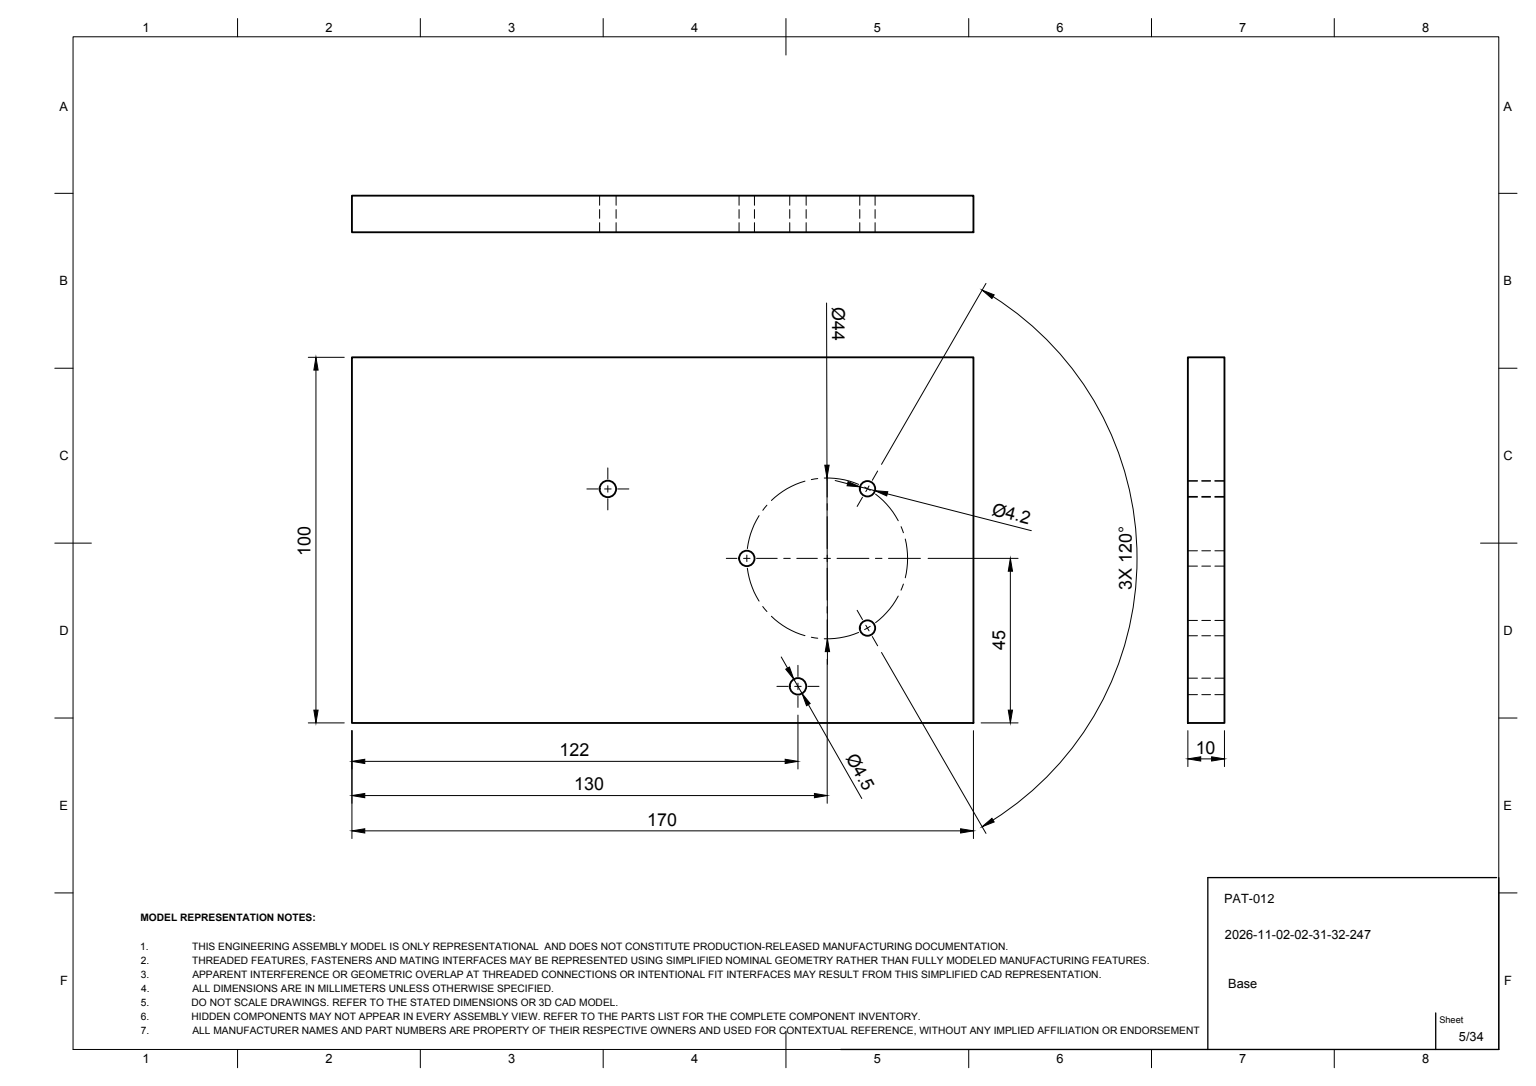
ISO-10303-21;
HEADER;
/* Generated by software containing ST-Developer
 * from STEP Tools, Inc. (www.steptools.com) 
 */

FILE_DESCRIPTION(
/* description */ ('Belt tensioner idler arm'),
/* implementation_level */ '2;1');

FILE_NAME(
/* name */ 'Base.step',
/* time_stamp */ '2026-10-28T03:22:15-07:00',
/* author */ (''),
/* organization */ (''),
/* preprocessor_version */ 'ST-DEVELOPER v20.2',
/* originating_system */ 'Autodesk Translation Framework v15.17.0.0',
/* authorisation */ '');

FILE_SCHEMA (('AUTOMOTIVE_DESIGN { 1 0 10303 214 3 1 1 }'));
ENDSEC;

DATA;
#10=MECHANICAL_DESIGN_GEOMETRIC_PRESENTATION_REPRESENTATION('',(#447),#12779);
#379=SHAPE_REPRESENTATION_RELATIONSHIP('SRR','None',#12925,#413);
#413=ADVANCED_BREP_SHAPE_REPRESENTATION('',(#489),#12742);
#447=STYLED_ITEM('',(#13163),#489);
#489=MANIFOLD_SOLID_BREP('Body1',#6181);
#527=FACE_BOUND('',#1214,.T.);
#528=FACE_BOUND('',#1215,.T.);
#529=FACE_BOUND('',#1216,.T.);
#530=FACE_BOUND('',#1217,.T.);
#531=FACE_BOUND('',#1218,.T.);
#532=FACE_BOUND('',#1220,.T.);
#533=FACE_BOUND('',#1221,.T.);
#534=FACE_BOUND('',#1222,.T.);
#535=FACE_BOUND('',#1223,.T.);
#536=FACE_BOUND('',#1224,.T.);
#663=PLANE('',#6620);
#664=PLANE('',#6621);
#665=PLANE('',#6622);
#666=PLANE('',#6623);
#667=PLANE('',#6624);
#668=PLANE('',#6625);
#837=FACE_OUTER_BOUND('',#1204,.T.);
#838=FACE_OUTER_BOUND('',#1205,.T.);
#839=FACE_OUTER_BOUND('',#1206,.T.);
#840=FACE_OUTER_BOUND('',#1207,.T.);
#841=FACE_OUTER_BOUND('',#1208,.T.);
#842=FACE_OUTER_BOUND('',#1209,.T.);
#843=FACE_OUTER_BOUND('',#1210,.T.);
#844=FACE_OUTER_BOUND('',#1211,.T.);
#845=FACE_OUTER_BOUND('',#1212,.T.);
#846=FACE_OUTER_BOUND('',#1213,.T.);
#847=FACE_OUTER_BOUND('',#1219,.T.);
#1204=EDGE_LOOP('',(#4086,#4087,#4088,#4089));
#1205=EDGE_LOOP('',(#4090,#4091,#4092,#4093));
#1206=EDGE_LOOP('',(#4094,#4095,#4096,#4097));
#1207=EDGE_LOOP('',(#4098,#4099,#4100,#4101));
#1208=EDGE_LOOP('',(#4102,#4103,#4104,#4105));
#1209=EDGE_LOOP('',(#4106,#4107,#4108,#4109));
#1210=EDGE_LOOP('',(#4110,#4111,#4112,#4113));
#1211=EDGE_LOOP('',(#4114,#4115,#4116,#4117));
#1212=EDGE_LOOP('',(#4118,#4119,#4120,#4121));
#1213=EDGE_LOOP('',(#4122,#4123,#4124,#4125));
#1214=EDGE_LOOP('',(#4126));
#1215=EDGE_LOOP('',(#4127));
#1216=EDGE_LOOP('',(#4128));
#1217=EDGE_LOOP('',(#4129));
#1218=EDGE_LOOP('',(#4130));
#1219=EDGE_LOOP('',(#4131,#4132,#4133,#4134));
#1220=EDGE_LOOP('',(#4135));
#1221=EDGE_LOOP('',(#4136));
#1222=EDGE_LOOP('',(#4137));
#1223=EDGE_LOOP('',(#4138));
#1224=EDGE_LOOP('',(#4139));
#1707=LINE('',#9451,#2056);
#1708=LINE('',#9457,#2057);
#1709=LINE('',#9463,#2058);
#1710=LINE('',#9469,#2059);
#1711=LINE('',#9475,#2060);
#1712=LINE('',#9480,#2061);
#1713=LINE('',#9482,#2062);
#1714=LINE('',#9484,#2063);
#1715=LINE('',#9485,#2064);
#1716=LINE('',#9488,#2065);
#1717=LINE('',#9490,#2066);
#1718=LINE('',#9491,#2067);
#1719=LINE('',#9494,#2068);
#1720=LINE('',#9496,#2069);
#1721=LINE('',#9497,#2070);
#1722=LINE('',#9499,#2071);
#1723=LINE('',#9500,#2072);
#2056=VECTOR('',#7443,0.225);
#2057=VECTOR('',#7450,0.225);
#2058=VECTOR('',#7457,0.21);
#2059=VECTOR('',#7464,0.21);
#2060=VECTOR('',#7471,0.21);
#2061=VECTOR('',#7476,1.);
#2062=VECTOR('',#7477,1.);
#2063=VECTOR('',#7478,1.);
#2064=VECTOR('',#7479,1.);
#2065=VECTOR('',#7482,1.);
#2066=VECTOR('',#7483,1.);
#2067=VECTOR('',#7484,1.);
#2068=VECTOR('',#7487,1.);
#2069=VECTOR('',#7488,1.);
#2070=VECTOR('',#7489,1.);
#2071=VECTOR('',#7492,1.);
#2072=VECTOR('',#7493,1.);
#2405=CIRCLE('',#6606,0.225);
#2406=CIRCLE('',#6607,0.225);
#2407=CIRCLE('',#6609,0.225);
#2408=CIRCLE('',#6610,0.225);
#2409=CIRCLE('',#6612,0.21);
#2410=CIRCLE('',#6613,0.21);
#2411=CIRCLE('',#6615,0.21);
#2412=CIRCLE('',#6616,0.21);
#2413=CIRCLE('',#6618,0.21);
#2414=CIRCLE('',#6619,0.21);
#2769=VERTEX_POINT('',#9448);
#2770=VERTEX_POINT('',#9450);
#2771=VERTEX_POINT('',#9454);
#2772=VERTEX_POINT('',#9456);
#2773=VERTEX_POINT('',#9460);
#2774=VERTEX_POINT('',#9462);
#2775=VERTEX_POINT('',#9466);
#2776=VERTEX_POINT('',#9468);
#2777=VERTEX_POINT('',#9472);
#2778=VERTEX_POINT('',#9474);
#2779=VERTEX_POINT('',#9478);
#2780=VERTEX_POINT('',#9479);
#2781=VERTEX_POINT('',#9481);
#2782=VERTEX_POINT('',#9483);
#2783=VERTEX_POINT('',#9487);
#2784=VERTEX_POINT('',#9489);
#2785=VERTEX_POINT('',#9493);
#2786=VERTEX_POINT('',#9495);
#3298=EDGE_CURVE('',#2769,#2769,#2405,.T.);
#3299=EDGE_CURVE('',#2769,#2770,#1707,.T.);
#3300=EDGE_CURVE('',#2770,#2770,#2406,.T.);
#3301=EDGE_CURVE('',#2771,#2771,#2407,.T.);
#3302=EDGE_CURVE('',#2771,#2772,#1708,.T.);
#3303=EDGE_CURVE('',#2772,#2772,#2408,.T.);
#3304=EDGE_CURVE('',#2773,#2773,#2409,.T.);
#3305=EDGE_CURVE('',#2773,#2774,#1709,.T.);
#3306=EDGE_CURVE('',#2774,#2774,#2410,.T.);
#3307=EDGE_CURVE('',#2775,#2775,#2411,.T.);
#3308=EDGE_CURVE('',#2775,#2776,#1710,.T.);
#3309=EDGE_CURVE('',#2776,#2776,#2412,.T.);
#3310=EDGE_CURVE('',#2777,#2777,#2413,.T.);
#3311=EDGE_CURVE('',#2777,#2778,#1711,.T.);
#3312=EDGE_CURVE('',#2778,#2778,#2414,.T.);
#3313=EDGE_CURVE('',#2779,#2780,#1712,.T.);
#3314=EDGE_CURVE('',#2780,#2781,#1713,.T.);
#3315=EDGE_CURVE('',#2782,#2781,#1714,.T.);
#3316=EDGE_CURVE('',#2779,#2782,#1715,.T.);
#3317=EDGE_CURVE('',#2783,#2779,#1716,.T.);
#3318=EDGE_CURVE('',#2784,#2782,#1717,.T.);
#3319=EDGE_CURVE('',#2783,#2784,#1718,.T.);
#3320=EDGE_CURVE('',#2785,#2783,#1719,.T.);
#3321=EDGE_CURVE('',#2786,#2784,#1720,.T.);
#3322=EDGE_CURVE('',#2785,#2786,#1721,.T.);
#3323=EDGE_CURVE('',#2780,#2785,#1722,.T.);
#3324=EDGE_CURVE('',#2781,#2786,#1723,.T.);
#4086=ORIENTED_EDGE('',*,*,#3298,.F.);
#4087=ORIENTED_EDGE('',*,*,#3299,.T.);
#4088=ORIENTED_EDGE('',*,*,#3300,.F.);
#4089=ORIENTED_EDGE('',*,*,#3299,.F.);
#4090=ORIENTED_EDGE('',*,*,#3301,.F.);
#4091=ORIENTED_EDGE('',*,*,#3302,.T.);
#4092=ORIENTED_EDGE('',*,*,#3303,.F.);
#4093=ORIENTED_EDGE('',*,*,#3302,.F.);
#4094=ORIENTED_EDGE('',*,*,#3304,.F.);
#4095=ORIENTED_EDGE('',*,*,#3305,.T.);
#4096=ORIENTED_EDGE('',*,*,#3306,.F.);
#4097=ORIENTED_EDGE('',*,*,#3305,.F.);
#4098=ORIENTED_EDGE('',*,*,#3307,.F.);
#4099=ORIENTED_EDGE('',*,*,#3308,.T.);
#4100=ORIENTED_EDGE('',*,*,#3309,.F.);
#4101=ORIENTED_EDGE('',*,*,#3308,.F.);
#4102=ORIENTED_EDGE('',*,*,#3310,.F.);
#4103=ORIENTED_EDGE('',*,*,#3311,.T.);
#4104=ORIENTED_EDGE('',*,*,#3312,.F.);
#4105=ORIENTED_EDGE('',*,*,#3311,.F.);
#4106=ORIENTED_EDGE('',*,*,#3313,.T.);
#4107=ORIENTED_EDGE('',*,*,#3314,.T.);
#4108=ORIENTED_EDGE('',*,*,#3315,.F.);
#4109=ORIENTED_EDGE('',*,*,#3316,.F.);
#4110=ORIENTED_EDGE('',*,*,#3317,.T.);
#4111=ORIENTED_EDGE('',*,*,#3316,.T.);
#4112=ORIENTED_EDGE('',*,*,#3318,.F.);
#4113=ORIENTED_EDGE('',*,*,#3319,.F.);
#4114=ORIENTED_EDGE('',*,*,#3320,.T.);
#4115=ORIENTED_EDGE('',*,*,#3319,.T.);
#4116=ORIENTED_EDGE('',*,*,#3321,.F.);
#4117=ORIENTED_EDGE('',*,*,#3322,.F.);
#4118=ORIENTED_EDGE('',*,*,#3323,.T.);
#4119=ORIENTED_EDGE('',*,*,#3322,.T.);
#4120=ORIENTED_EDGE('',*,*,#3324,.F.);
#4121=ORIENTED_EDGE('',*,*,#3314,.F.);
#4122=ORIENTED_EDGE('',*,*,#3324,.T.);
#4123=ORIENTED_EDGE('',*,*,#3321,.T.);
#4124=ORIENTED_EDGE('',*,*,#3318,.T.);
#4125=ORIENTED_EDGE('',*,*,#3315,.T.);
#4126=ORIENTED_EDGE('',*,*,#3300,.T.);
#4127=ORIENTED_EDGE('',*,*,#3303,.T.);
#4128=ORIENTED_EDGE('',*,*,#3306,.T.);
#4129=ORIENTED_EDGE('',*,*,#3309,.T.);
#4130=ORIENTED_EDGE('',*,*,#3312,.T.);
#4131=ORIENTED_EDGE('',*,*,#3323,.F.);
#4132=ORIENTED_EDGE('',*,*,#3313,.F.);
#4133=ORIENTED_EDGE('',*,*,#3317,.F.);
#4134=ORIENTED_EDGE('',*,*,#3320,.F.);
#4135=ORIENTED_EDGE('',*,*,#3298,.T.);
#4136=ORIENTED_EDGE('',*,*,#3301,.T.);
#4137=ORIENTED_EDGE('',*,*,#3304,.T.);
#4138=ORIENTED_EDGE('',*,*,#3307,.T.);
#4139=ORIENTED_EDGE('',*,*,#3310,.T.);
#5662=CYLINDRICAL_SURFACE('',#6605,0.225);
#5663=CYLINDRICAL_SURFACE('',#6608,0.225);
#5664=CYLINDRICAL_SURFACE('',#6611,0.21);
#5665=CYLINDRICAL_SURFACE('',#6614,0.21);
#5666=CYLINDRICAL_SURFACE('',#6617,0.21);
#5814=ADVANCED_FACE('',(#837),#5662,.F.);
#5815=ADVANCED_FACE('',(#838),#5663,.F.);
#5816=ADVANCED_FACE('',(#839),#5664,.F.);
#5817=ADVANCED_FACE('',(#840),#5665,.F.);
#5818=ADVANCED_FACE('',(#841),#5666,.F.);
#5819=ADVANCED_FACE('',(#842),#663,.T.);
#5820=ADVANCED_FACE('',(#843),#664,.T.);
#5821=ADVANCED_FACE('',(#844),#665,.T.);
#5822=ADVANCED_FACE('',(#845),#666,.T.);
#5823=ADVANCED_FACE('',(#846,#527,#528,#529,#530,#531),#667,.T.);
#5824=ADVANCED_FACE('',(#847,#532,#533,#534,#535,#536),#668,.F.);
#6181=CLOSED_SHELL('',(#5814,#5815,#5816,#5817,#5818,#5819,#5820,#5821,
#5822,#5823,#5824));
#6604=AXIS2_PLACEMENT_3D('',#9446,#7437,#7438);
#6605=AXIS2_PLACEMENT_3D('',#9447,#7439,#7440);
#6606=AXIS2_PLACEMENT_3D('',#9449,#7441,#7442);
#6607=AXIS2_PLACEMENT_3D('',#9452,#7444,#7445);
#6608=AXIS2_PLACEMENT_3D('',#9453,#7446,#7447);
#6609=AXIS2_PLACEMENT_3D('',#9455,#7448,#7449);
#6610=AXIS2_PLACEMENT_3D('',#9458,#7451,#7452);
#6611=AXIS2_PLACEMENT_3D('',#9459,#7453,#7454);
#6612=AXIS2_PLACEMENT_3D('',#9461,#7455,#7456);
#6613=AXIS2_PLACEMENT_3D('',#9464,#7458,#7459);
#6614=AXIS2_PLACEMENT_3D('',#9465,#7460,#7461);
#6615=AXIS2_PLACEMENT_3D('',#9467,#7462,#7463);
#6616=AXIS2_PLACEMENT_3D('',#9470,#7465,#7466);
#6617=AXIS2_PLACEMENT_3D('',#9471,#7467,#7468);
#6618=AXIS2_PLACEMENT_3D('',#9473,#7469,#7470);
#6619=AXIS2_PLACEMENT_3D('',#9476,#7472,#7473);
#6620=AXIS2_PLACEMENT_3D('',#9477,#7474,#7475);
#6621=AXIS2_PLACEMENT_3D('',#9486,#7480,#7481);
#6622=AXIS2_PLACEMENT_3D('',#9492,#7485,#7486);
#6623=AXIS2_PLACEMENT_3D('',#9498,#7490,#7491);
#6624=AXIS2_PLACEMENT_3D('',#9501,#7494,#7495);
#6625=AXIS2_PLACEMENT_3D('',#9502,#7496,#7497);
#7437=DIRECTION('axis',(0.,0.,1.));
#7438=DIRECTION('refdir',(1.,0.,0.));
#7439=DIRECTION('center_axis',(0.,0.,1.));
#7440=DIRECTION('ref_axis',(1.,0.,0.));
#7441=DIRECTION('center_axis',(0.,0.,1.));
#7442=DIRECTION('ref_axis',(1.,0.,0.));
#7443=DIRECTION('',(0.,0.,1.));
#7444=DIRECTION('center_axis',(0.,0.,-1.));
#7445=DIRECTION('ref_axis',(1.,0.,0.));
#7446=DIRECTION('center_axis',(0.,0.,1.));
#7447=DIRECTION('ref_axis',(1.,0.,0.));
#7448=DIRECTION('center_axis',(0.,0.,1.));
#7449=DIRECTION('ref_axis',(1.,0.,0.));
#7450=DIRECTION('',(0.,0.,1.));
#7451=DIRECTION('center_axis',(0.,0.,-1.));
#7452=DIRECTION('ref_axis',(1.,0.,0.));
#7453=DIRECTION('center_axis',(0.,0.,1.));
#7454=DIRECTION('ref_axis',(1.,0.,0.));
#7455=DIRECTION('center_axis',(0.,0.,1.));
#7456=DIRECTION('ref_axis',(1.,0.,0.));
#7457=DIRECTION('',(0.,0.,1.));
#7458=DIRECTION('center_axis',(0.,0.,-1.));
#7459=DIRECTION('ref_axis',(1.,0.,0.));
#7460=DIRECTION('center_axis',(0.,0.,1.));
#7461=DIRECTION('ref_axis',(1.,0.,0.));
#7462=DIRECTION('center_axis',(0.,0.,1.));
#7463=DIRECTION('ref_axis',(1.,0.,0.));
#7464=DIRECTION('',(0.,0.,1.));
#7465=DIRECTION('center_axis',(0.,0.,-1.));
#7466=DIRECTION('ref_axis',(1.,0.,0.));
#7467=DIRECTION('center_axis',(0.,0.,1.));
#7468=DIRECTION('ref_axis',(1.,0.,0.));
#7469=DIRECTION('center_axis',(0.,0.,1.));
#7470=DIRECTION('ref_axis',(1.,0.,0.));
#7471=DIRECTION('',(0.,0.,1.));
#7472=DIRECTION('center_axis',(0.,0.,-1.));
#7473=DIRECTION('ref_axis',(1.,0.,0.));
#7474=DIRECTION('center_axis',(0.,1.,0.));
#7475=DIRECTION('ref_axis',(-1.,0.,0.));
#7476=DIRECTION('',(-1.,0.,0.));
#7477=DIRECTION('',(0.,0.,1.));
#7478=DIRECTION('',(-1.,0.,0.));
#7479=DIRECTION('',(0.,0.,1.));
#7480=DIRECTION('center_axis',(1.,0.,0.));
#7481=DIRECTION('ref_axis',(0.,1.,0.));
#7482=DIRECTION('',(0.,1.,0.));
#7483=DIRECTION('',(0.,1.,0.));
#7484=DIRECTION('',(0.,0.,1.));
#7485=DIRECTION('center_axis',(0.,-1.,0.));
#7486=DIRECTION('ref_axis',(1.,0.,0.));
#7487=DIRECTION('',(1.,0.,0.));
#7488=DIRECTION('',(1.,0.,0.));
#7489=DIRECTION('',(0.,0.,1.));
#7490=DIRECTION('center_axis',(-1.,0.,0.));
#7491=DIRECTION('ref_axis',(0.,-1.,0.));
#7492=DIRECTION('',(0.,-1.,0.));
#7493=DIRECTION('',(0.,-1.,0.));
#7494=DIRECTION('center_axis',(0.,0.,1.));
#7495=DIRECTION('ref_axis',(1.,0.,0.));
#7496=DIRECTION('center_axis',(0.,0.,1.));
#7497=DIRECTION('ref_axis',(1.,0.,0.));
#9446=CARTESIAN_POINT('',(0.,0.,0.));
#9447=CARTESIAN_POINT('Origin',(6.,1.9,-1.1));
#9448=CARTESIAN_POINT('',(5.775,1.9,-1.));
#9449=CARTESIAN_POINT('Origin',(6.,1.9,-1.));
#9450=CARTESIAN_POINT('',(5.775,1.9,0.));
#9451=CARTESIAN_POINT('',(5.775,1.9,-1.1));
#9452=CARTESIAN_POINT('Origin',(6.,1.9,0.));
#9453=CARTESIAN_POINT('Origin',(0.8,-3.5,-1.1));
#9454=CARTESIAN_POINT('',(0.575,-3.5,-1.));
#9455=CARTESIAN_POINT('Origin',(0.8,-3.5,-1.));
#9456=CARTESIAN_POINT('',(0.575,-3.5,0.));
#9457=CARTESIAN_POINT('',(0.575,-3.5,-1.1));
#9458=CARTESIAN_POINT('Origin',(0.8,-3.5,0.));
#9459=CARTESIAN_POINT('Origin',(2.2,0.,-1.1));
#9460=CARTESIAN_POINT('',(1.99,-2.57175827820944E-17,-1.));
#9461=CARTESIAN_POINT('Origin',(2.2,0.,-1.));
#9462=CARTESIAN_POINT('',(1.99,2.57175827820944E-17,0.));
#9463=CARTESIAN_POINT('',(1.99,-2.57175827820944E-17,-1.1));
#9464=CARTESIAN_POINT('Origin',(2.2,0.,0.));
#9465=CARTESIAN_POINT('Origin',(-1.1,1.90525588832577,-1.1));
#9466=CARTESIAN_POINT('',(-1.31,1.90525588832577,-1.));
#9467=CARTESIAN_POINT('Origin',(-1.1,1.90525588832577,-1.));
#9468=CARTESIAN_POINT('',(-1.31,1.90525588832577,0.));
#9469=CARTESIAN_POINT('',(-1.31,1.90525588832577,-1.1));
#9470=CARTESIAN_POINT('Origin',(-1.1,1.90525588832577,0.));
#9471=CARTESIAN_POINT('Origin',(-1.1,-1.90525588832576,-1.1));
#9472=CARTESIAN_POINT('',(-1.31,-1.90525588832576,-1.));
#9473=CARTESIAN_POINT('Origin',(-1.1,-1.90525588832576,-1.));
#9474=CARTESIAN_POINT('',(-1.31,-1.90525588832576,0.));
#9475=CARTESIAN_POINT('',(-1.31,-1.90525588832576,-1.1));
#9476=CARTESIAN_POINT('Origin',(-1.1,-1.90525588832576,0.));
#9477=CARTESIAN_POINT('Origin',(13.,5.5,-1.));
#9478=CARTESIAN_POINT('',(13.,5.5,-1.));
#9479=CARTESIAN_POINT('',(-4.,5.5,-1.));
#9480=CARTESIAN_POINT('',(13.,5.5,-1.));
#9481=CARTESIAN_POINT('',(-4.,5.5,0.));
#9482=CARTESIAN_POINT('',(-4.,5.5,-1.));
#9483=CARTESIAN_POINT('',(13.,5.5,0.));
#9484=CARTESIAN_POINT('',(13.,5.5,0.));
#9485=CARTESIAN_POINT('',(13.,5.5,-1.));
#9486=CARTESIAN_POINT('Origin',(13.,-4.5,-1.));
#9487=CARTESIAN_POINT('',(13.,-4.5,-1.));
#9488=CARTESIAN_POINT('',(13.,-4.5,-1.));
#9489=CARTESIAN_POINT('',(13.,-4.5,0.));
#9490=CARTESIAN_POINT('',(13.,-4.5,0.));
#9491=CARTESIAN_POINT('',(13.,-4.5,-1.));
#9492=CARTESIAN_POINT('Origin',(-4.,-4.5,-1.));
#9493=CARTESIAN_POINT('',(-4.,-4.5,-1.));
#9494=CARTESIAN_POINT('',(-4.,-4.5,-1.));
#9495=CARTESIAN_POINT('',(-4.,-4.5,0.));
#9496=CARTESIAN_POINT('',(-4.,-4.5,0.));
#9497=CARTESIAN_POINT('',(-4.,-4.5,-1.));
#9498=CARTESIAN_POINT('Origin',(-4.,5.5,-1.));
#9499=CARTESIAN_POINT('',(-4.,5.5,-1.));
#9500=CARTESIAN_POINT('',(-4.,5.5,0.));
#9501=CARTESIAN_POINT('Origin',(4.5,0.5,0.));
#9502=CARTESIAN_POINT('Origin',(4.5,0.5,-1.));
#12702=UNCERTAINTY_MEASURE_WITH_UNIT(LENGTH_MEASURE(0.001),#12780,
'DISTANCE_ACCURACY_VALUE',
'Maximum model space distance between geometric entities at asserted c
onnectivities');
#12739=UNCERTAINTY_MEASURE_WITH_UNIT(LENGTH_MEASURE(0.001),#12780,
'DISTANCE_ACCURACY_VALUE',
'Maximum model space distance between geometric entities at asserted c
onnectivities');
#12742=(
GEOMETRIC_REPRESENTATION_CONTEXT(3)
GLOBAL_UNCERTAINTY_ASSIGNED_CONTEXT((#12702))
GLOBAL_UNIT_ASSIGNED_CONTEXT((#12780,#12782,#12783))
REPRESENTATION_CONTEXT('','3D')
);
#12779=(
GEOMETRIC_REPRESENTATION_CONTEXT(3)
GLOBAL_UNCERTAINTY_ASSIGNED_CONTEXT((#12739))
GLOBAL_UNIT_ASSIGNED_CONTEXT((#12780,#12782,#12783))
REPRESENTATION_CONTEXT('','3D')
);
#12780=(
LENGTH_UNIT()
NAMED_UNIT(*)
SI_UNIT(.CENTI.,.METRE.)
);
#12782=(
NAMED_UNIT(*)
PLANE_ANGLE_UNIT()
SI_UNIT($,.RADIAN.)
);
#12783=(
NAMED_UNIT(*)
SI_UNIT($,.STERADIAN.)
SOLID_ANGLE_UNIT()
);
#12786=SHAPE_DEFINITION_REPRESENTATION(#12825,#12925);
#12825=PRODUCT_DEFINITION_SHAPE('',$,#12965);
#12925=SHAPE_REPRESENTATION('',(#6604),#12742);
#12962=PRODUCT_DEFINITION_CONTEXT('part definition',#13081,'design');
#12965=PRODUCT_DEFINITION('Base','Base',#13004,#12962);
#13004=PRODUCT_DEFINITION_FORMATION('',$,#13085);
#13081=APPLICATION_CONTEXT(
'Core Data for Automotive Mechanical Design Process');
#13082=PRODUCT_CONTEXT('part definition',#13081,'mechanical');
#13085=PRODUCT('Base','Base','Base',(#13082));
#13157=COLOUR_RGB('Dark Blue',0.08,0.2,0.34);
#13158=FILL_AREA_STYLE_COLOUR('',#13157);
#13159=FILL_AREA_STYLE('',(#13158));
#13160=SURFACE_STYLE_FILL_AREA(#13159);
#13161=SURFACE_SIDE_STYLE('',(#13160));
#13162=SURFACE_STYLE_USAGE(.BOTH.,#13161);
#13163=PRESENTATION_STYLE_ASSIGNMENT((#13162));
ENDSEC;
END-ISO-10303-21;
